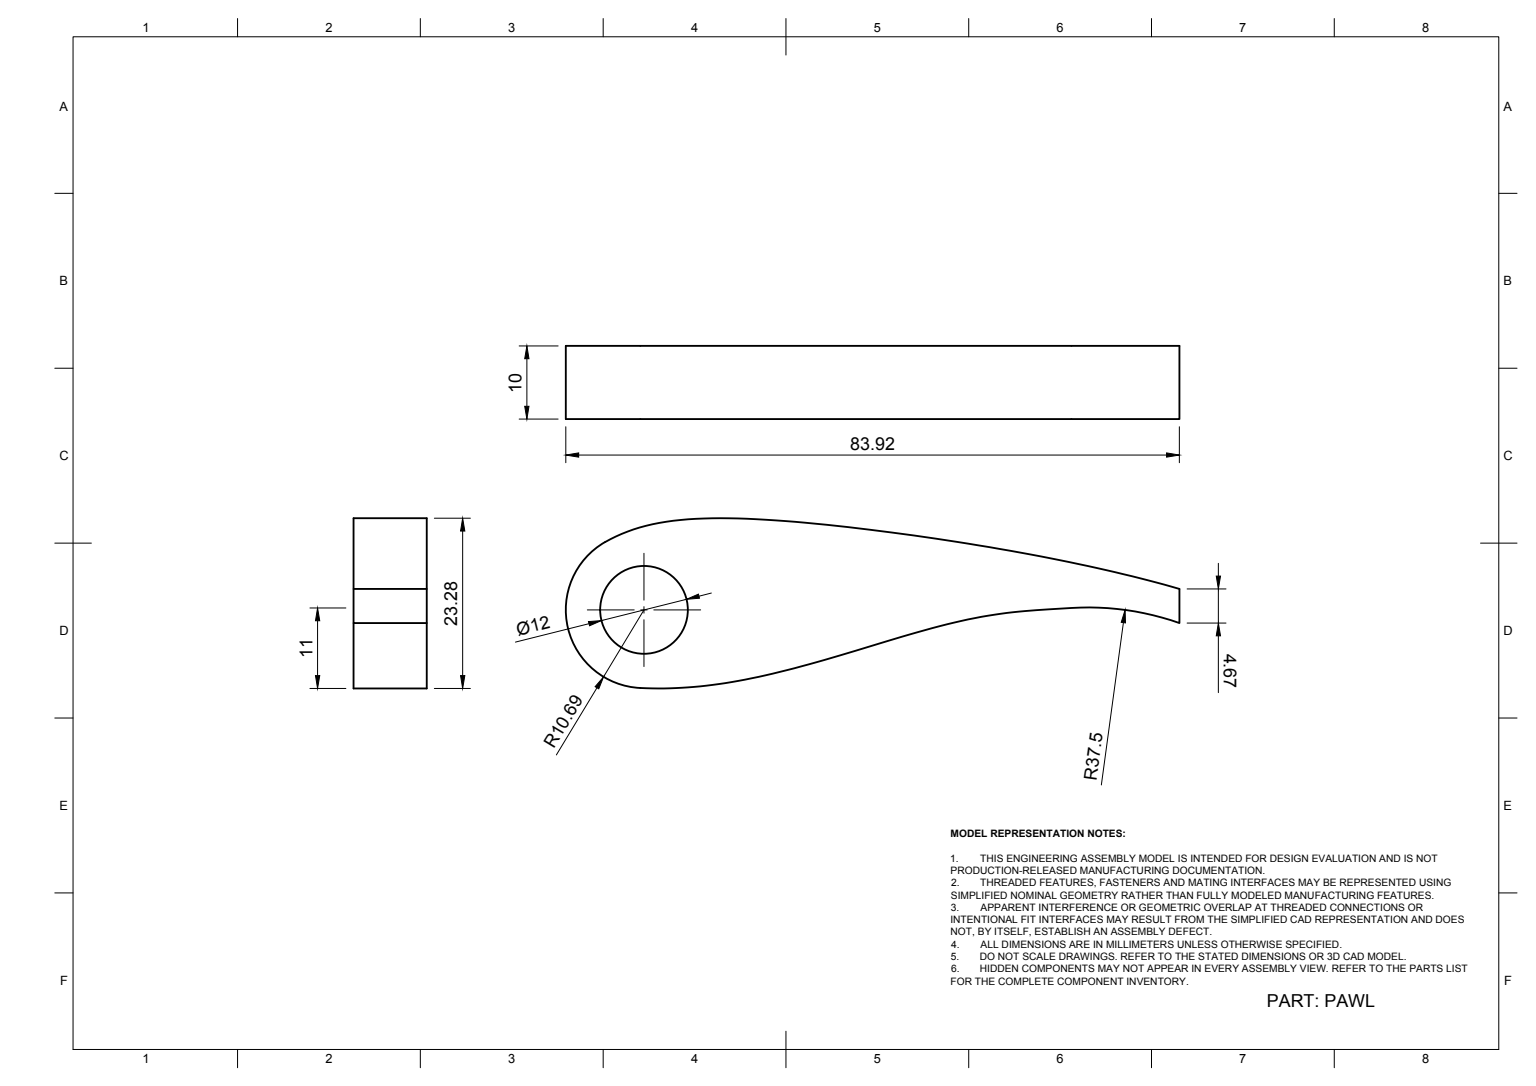
ISO-10303-21;
HEADER;
/* Generated by software containing ST-Developer
 * from STEP Tools, Inc. (www.steptools.com) 
 */

FILE_DESCRIPTION(
/* description */ (''),
/* implementation_level */ '2;1');

FILE_NAME(
/* name */ 'Pawl.step',
/* time_stamp */ '2026-09-20T22:38:01+06:00',
/* author */ (''),
/* organization */ (''),
/* preprocessor_version */ 'ST-DEVELOPER v20.2',
/* originating_system */ 'Autodesk Translation Framework v15.15.0.0',
/* authorisation */ '');

FILE_SCHEMA (('AUTOMOTIVE_DESIGN { 1 0 10303 214 3 1 1 }'));
ENDSEC;

DATA;
#10=MECHANICAL_DESIGN_GEOMETRIC_PRESENTATION_REPRESENTATION('',(#85),#4079);
#62=(
BOUNDED_CURVE()
B_SPLINE_CURVE(5,(#2402,#2403,#2404,#2405,#2406,#2407,#2408,#2409,#2410,
#2411,#2412,#2413,#2414,#2415,#2416,#2417,#2418,#2419,#2420,#2421),
 .UNSPECIFIED.,.F.,.F.)
B_SPLINE_CURVE_WITH_KNOTS((6,1,1,1,1,1,1,1,1,1,1,1,1,1,1,6),(0.,0.0666666666666667,
0.133333333333333,0.2,0.266666666666667,0.333333333333333,0.4,0.466666666666667,
0.533333333333333,0.6,0.666666666666667,0.733333333333333,0.8,0.866666666666667,
0.933333333333333,1.),.UNSPECIFIED.)
CURVE()
GEOMETRIC_REPRESENTATION_ITEM()
RATIONAL_B_SPLINE_CURVE((1.,1.,1.,1.,1.,1.,1.,1.,1.,1.,1.,1.,1.,1.,1.,1.,
1.,1.,1.,1.))
REPRESENTATION_ITEM('')
);
#63=(
BOUNDED_CURVE()
B_SPLINE_CURVE(5,(#2425,#2426,#2427,#2428,#2429,#2430,#2431,#2432,#2433,
#2434,#2435,#2436,#2437,#2438,#2439,#2440,#2441,#2442,#2443,#2444),
 .UNSPECIFIED.,.F.,.F.)
B_SPLINE_CURVE_WITH_KNOTS((6,1,1,1,1,1,1,1,1,1,1,1,1,1,1,6),(-1.,-0.933333333333333,
-0.866666666666667,-0.8,-0.733333333333333,-0.666666666666667,-0.6,-0.533333333333333,
-0.466666666666667,-0.4,-0.333333333333333,-0.266666666666667,-0.2,-0.133333333333333,
-0.0666666666666667,0.),.UNSPECIFIED.)
CURVE()
GEOMETRIC_REPRESENTATION_ITEM()
RATIONAL_B_SPLINE_CURVE((1.,1.,1.,1.,1.,1.,1.,1.,1.,1.,1.,1.,1.,1.,1.,1.,
1.,1.,1.,1.))
REPRESENTATION_ITEM('')
);
#64=(
BOUNDED_CURVE()
B_SPLINE_CURVE(5,(#2503,#2504,#2505,#2506,#2507,#2508,#2509,#2510,#2511,
#2512,#2513,#2514,#2515,#2516,#2517,#2518,#2519,#2520,#2521,#2522,#2523,
#2524,#2525,#2526,#2527),.UNSPECIFIED.,.F.,.F.)
B_SPLINE_CURVE_WITH_KNOTS((6,1,1,1,1,1,1,1,1,1,1,1,1,1,1,1,1,1,1,1,6),(0.,
0.05,0.1,0.15,0.2,0.25,0.3,0.35,0.4,0.45,0.5,0.55,0.6,0.65,0.7,0.75,0.8,
0.85,0.9,0.95,1.),.UNSPECIFIED.)
CURVE()
GEOMETRIC_REPRESENTATION_ITEM()
RATIONAL_B_SPLINE_CURVE((1.,1.,1.,1.,1.,1.,1.,1.,1.,1.,1.,1.,1.,1.,1.,1.,
1.,1.,1.,1.,1.,1.,1.,1.,1.))
REPRESENTATION_ITEM('')
);
#65=(
BOUNDED_CURVE()
B_SPLINE_CURVE(5,(#2529,#2530,#2531,#2532,#2533,#2534,#2535,#2536,#2537,
#2538,#2539,#2540,#2541,#2542,#2543,#2544,#2545,#2546,#2547,#2548,#2549,
#2550,#2551,#2552,#2553),.UNSPECIFIED.,.F.,.F.)
B_SPLINE_CURVE_WITH_KNOTS((6,1,1,1,1,1,1,1,1,1,1,1,1,1,1,1,1,1,1,1,6),(0.,
0.05,0.1,0.15,0.2,0.25,0.3,0.35,0.4,0.45,0.5,0.55,0.6,0.65,0.7,0.75,0.8,
0.85,0.9,0.95,1.),.UNSPECIFIED.)
CURVE()
GEOMETRIC_REPRESENTATION_ITEM()
RATIONAL_B_SPLINE_CURVE((1.,1.,1.,1.,1.,1.,1.,1.,1.,1.,1.,1.,1.,1.,1.,1.,
1.,1.,1.,1.,1.,1.,1.,1.,1.))
REPRESENTATION_ITEM('')
);
#66=(
BOUNDED_SURFACE()
B_SPLINE_SURFACE(5,1,((#2360,#2361),(#2362,#2363),(#2364,#2365),(#2366,
#2367),(#2368,#2369),(#2370,#2371),(#2372,#2373),(#2374,#2375),(#2376,#2377),
(#2378,#2379),(#2380,#2381),(#2382,#2383),(#2384,#2385),(#2386,#2387),(#2388,
#2389),(#2390,#2391),(#2392,#2393),(#2394,#2395),(#2396,#2397),(#2398,#2399)),
 .UNSPECIFIED.,.F.,.F.,.F.)
B_SPLINE_SURFACE_WITH_KNOTS((6,1,1,1,1,1,1,1,1,1,1,1,1,1,1,6),(2,2),(-1.,
-0.933333333333333,-0.866666666666667,-0.8,-0.733333333333333,-0.666666666666667,
-0.6,-0.533333333333333,-0.466666666666667,-0.4,-0.333333333333333,-0.266666666666667,
-0.2,-0.133333333333333,-0.0666666666666667,0.),(0.,1.),.UNSPECIFIED.)
GEOMETRIC_REPRESENTATION_ITEM()
RATIONAL_B_SPLINE_SURFACE(((1.,1.),(1.,1.),(1.,1.),(1.,1.),(1.,1.),(1.,
1.),(1.,1.),(1.,1.),(1.,1.),(1.,1.),(1.,1.),(1.,1.),(1.,1.),(1.,1.),(1.,
1.),(1.,1.),(1.,1.),(1.,1.),(1.,1.),(1.,1.)))
REPRESENTATION_ITEM('')
SURFACE()
);
#67=(
BOUNDED_SURFACE()
B_SPLINE_SURFACE(5,1,((#2452,#2453),(#2454,#2455),(#2456,#2457),(#2458,
#2459),(#2460,#2461),(#2462,#2463),(#2464,#2465),(#2466,#2467),(#2468,#2469),
(#2470,#2471),(#2472,#2473),(#2474,#2475),(#2476,#2477),(#2478,#2479),(#2480,
#2481),(#2482,#2483),(#2484,#2485),(#2486,#2487),(#2488,#2489),(#2490,#2491),
(#2492,#2493),(#2494,#2495),(#2496,#2497),(#2498,#2499),(#2500,#2501)),
 .UNSPECIFIED.,.F.,.F.,.F.)
B_SPLINE_SURFACE_WITH_KNOTS((6,1,1,1,1,1,1,1,1,1,1,1,1,1,1,1,1,1,1,1,6),
(2,2),(0.,0.05,0.1,0.15,0.2,0.25,0.3,0.35,0.4,0.45,0.5,0.55,0.6,0.65,0.7,
0.75,0.8,0.85,0.9,0.95,1.),(0.,1.),.UNSPECIFIED.)
GEOMETRIC_REPRESENTATION_ITEM()
RATIONAL_B_SPLINE_SURFACE(((1.,1.),(1.,1.),(1.,1.),(1.,1.),(1.,1.),(1.,
1.),(1.,1.),(1.,1.),(1.,1.),(1.,1.),(1.,1.),(1.,1.),(1.,1.),(1.,1.),(1.,
1.),(1.,1.),(1.,1.),(1.,1.),(1.,1.),(1.,1.),(1.,1.),(1.,1.),(1.,1.),(1.,
1.),(1.,1.)))
REPRESENTATION_ITEM('')
SURFACE()
);
#69=SHAPE_REPRESENTATION_RELATIONSHIP('SRR','None',#4112,#77);
#77=ADVANCED_BREP_SHAPE_REPRESENTATION('',(#93),#4072);
#85=STYLED_ITEM('',(#4161),#93);
#93=MANIFOLD_SOLID_BREP('Pawl',#1444);
#102=FACE_BOUND('',#329,.T.);
#103=FACE_BOUND('',#331,.T.);
#144=CIRCLE('',#1621,6.);
#145=CIRCLE('',#1622,6.);
#146=CIRCLE('',#1624,10.6886401797172);
#147=CIRCLE('',#1625,10.6886401797172);
#148=CIRCLE('',#1627,37.4987147312738);
#149=CIRCLE('',#1628,37.4987147312738);
#188=CYLINDRICAL_SURFACE('',#1620,6.);
#189=CYLINDRICAL_SURFACE('',#1623,10.6886401797172);
#190=CYLINDRICAL_SURFACE('',#1626,37.4987147312738);
#236=FACE_OUTER_BOUND('',#322,.T.);
#237=FACE_OUTER_BOUND('',#323,.T.);
#238=FACE_OUTER_BOUND('',#324,.T.);
#239=FACE_OUTER_BOUND('',#325,.T.);
#240=FACE_OUTER_BOUND('',#326,.T.);
#241=FACE_OUTER_BOUND('',#327,.T.);
#242=FACE_OUTER_BOUND('',#328,.T.);
#243=FACE_OUTER_BOUND('',#330,.T.);
#322=EDGE_LOOP('',(#1141,#1142,#1143,#1144));
#323=EDGE_LOOP('',(#1145,#1146,#1147,#1148));
#324=EDGE_LOOP('',(#1149,#1150,#1151,#1152));
#325=EDGE_LOOP('',(#1153,#1154,#1155,#1156));
#326=EDGE_LOOP('',(#1157,#1158,#1159,#1160));
#327=EDGE_LOOP('',(#1161,#1162,#1163,#1164));
#328=EDGE_LOOP('',(#1165,#1166,#1167,#1168,#1169));
#329=EDGE_LOOP('',(#1170));
#330=EDGE_LOOP('',(#1171,#1172,#1173,#1174,#1175));
#331=EDGE_LOOP('',(#1176));
#444=LINE('',#2358,#557);
#445=LINE('',#2423,#558);
#446=LINE('',#2445,#559);
#447=LINE('',#2451,#560);
#448=LINE('',#2554,#561);
#449=LINE('',#2560,#562);
#450=LINE('',#2562,#563);
#451=LINE('',#2563,#564);
#557=VECTOR('',#1935,6.);
#558=VECTOR('',#1938,10.);
#559=VECTOR('',#1939,10.);
#560=VECTOR('',#1946,10.);
#561=VECTOR('',#1947,10.);
#562=VECTOR('',#1954,10.);
#563=VECTOR('',#1957,10.);
#564=VECTOR('',#1958,10.);
#671=VERTEX_POINT('',#2355);
#672=VERTEX_POINT('',#2357);
#673=VERTEX_POINT('',#2400);
#674=VERTEX_POINT('',#2401);
#675=VERTEX_POINT('',#2422);
#676=VERTEX_POINT('',#2424);
#677=VERTEX_POINT('',#2447);
#678=VERTEX_POINT('',#2449);
#679=VERTEX_POINT('',#2502);
#680=VERTEX_POINT('',#2528);
#681=VERTEX_POINT('',#2556);
#682=VERTEX_POINT('',#2558);
#835=EDGE_CURVE('',#671,#671,#144,.T.);
#836=EDGE_CURVE('',#671,#672,#444,.T.);
#837=EDGE_CURVE('',#672,#672,#145,.T.);
#838=EDGE_CURVE('',#673,#674,#62,.T.);
#839=EDGE_CURVE('',#673,#675,#445,.T.);
#840=EDGE_CURVE('',#676,#675,#63,.T.);
#841=EDGE_CURVE('',#674,#676,#446,.T.);
#842=EDGE_CURVE('',#674,#677,#146,.T.);
#843=EDGE_CURVE('',#678,#676,#147,.T.);
#844=EDGE_CURVE('',#677,#678,#447,.T.);
#845=EDGE_CURVE('',#679,#677,#64,.T.);
#846=EDGE_CURVE('',#680,#678,#65,.T.);
#847=EDGE_CURVE('',#679,#680,#448,.T.);
#848=EDGE_CURVE('',#681,#679,#148,.T.);
#849=EDGE_CURVE('',#682,#680,#149,.T.);
#850=EDGE_CURVE('',#681,#682,#449,.T.);
#851=EDGE_CURVE('',#681,#673,#450,.T.);
#852=EDGE_CURVE('',#675,#682,#451,.T.);
#1141=ORIENTED_EDGE('',*,*,#835,.F.);
#1142=ORIENTED_EDGE('',*,*,#836,.T.);
#1143=ORIENTED_EDGE('',*,*,#837,.F.);
#1144=ORIENTED_EDGE('',*,*,#836,.F.);
#1145=ORIENTED_EDGE('',*,*,#838,.F.);
#1146=ORIENTED_EDGE('',*,*,#839,.T.);
#1147=ORIENTED_EDGE('',*,*,#840,.F.);
#1148=ORIENTED_EDGE('',*,*,#841,.F.);
#1149=ORIENTED_EDGE('',*,*,#842,.F.);
#1150=ORIENTED_EDGE('',*,*,#841,.T.);
#1151=ORIENTED_EDGE('',*,*,#843,.F.);
#1152=ORIENTED_EDGE('',*,*,#844,.F.);
#1153=ORIENTED_EDGE('',*,*,#845,.T.);
#1154=ORIENTED_EDGE('',*,*,#844,.T.);
#1155=ORIENTED_EDGE('',*,*,#846,.F.);
#1156=ORIENTED_EDGE('',*,*,#847,.F.);
#1157=ORIENTED_EDGE('',*,*,#848,.T.);
#1158=ORIENTED_EDGE('',*,*,#847,.T.);
#1159=ORIENTED_EDGE('',*,*,#849,.F.);
#1160=ORIENTED_EDGE('',*,*,#850,.F.);
#1161=ORIENTED_EDGE('',*,*,#851,.F.);
#1162=ORIENTED_EDGE('',*,*,#850,.T.);
#1163=ORIENTED_EDGE('',*,*,#852,.F.);
#1164=ORIENTED_EDGE('',*,*,#839,.F.);
#1165=ORIENTED_EDGE('',*,*,#851,.T.);
#1166=ORIENTED_EDGE('',*,*,#838,.T.);
#1167=ORIENTED_EDGE('',*,*,#842,.T.);
#1168=ORIENTED_EDGE('',*,*,#845,.F.);
#1169=ORIENTED_EDGE('',*,*,#848,.F.);
#1170=ORIENTED_EDGE('',*,*,#835,.T.);
#1171=ORIENTED_EDGE('',*,*,#852,.T.);
#1172=ORIENTED_EDGE('',*,*,#849,.T.);
#1173=ORIENTED_EDGE('',*,*,#846,.T.);
#1174=ORIENTED_EDGE('',*,*,#843,.T.);
#1175=ORIENTED_EDGE('',*,*,#840,.T.);
#1176=ORIENTED_EDGE('',*,*,#837,.T.);
#1329=PLANE('',#1629);
#1330=PLANE('',#1630);
#1331=PLANE('',#1631);
#1398=ADVANCED_FACE('',(#236),#188,.F.);
#1399=ADVANCED_FACE('',(#237),#66,.T.);
#1400=ADVANCED_FACE('',(#238),#189,.T.);
#1401=ADVANCED_FACE('',(#239),#67,.T.);
#1402=ADVANCED_FACE('',(#240),#190,.F.);
#1403=ADVANCED_FACE('',(#241),#1329,.T.);
#1404=ADVANCED_FACE('',(#242,#102),#1330,.T.);
#1405=ADVANCED_FACE('',(#243,#103),#1331,.F.);
#1444=CLOSED_SHELL('',(#1398,#1399,#1400,#1401,#1402,#1403,#1404,#1405));
#1619=AXIS2_PLACEMENT_3D('',#2353,#1929,#1930);
#1620=AXIS2_PLACEMENT_3D('',#2354,#1931,#1932);
#1621=AXIS2_PLACEMENT_3D('',#2356,#1933,#1934);
#1622=AXIS2_PLACEMENT_3D('',#2359,#1936,#1937);
#1623=AXIS2_PLACEMENT_3D('',#2446,#1940,#1941);
#1624=AXIS2_PLACEMENT_3D('',#2448,#1942,#1943);
#1625=AXIS2_PLACEMENT_3D('',#2450,#1944,#1945);
#1626=AXIS2_PLACEMENT_3D('',#2555,#1948,#1949);
#1627=AXIS2_PLACEMENT_3D('',#2557,#1950,#1951);
#1628=AXIS2_PLACEMENT_3D('',#2559,#1952,#1953);
#1629=AXIS2_PLACEMENT_3D('',#2561,#1955,#1956);
#1630=AXIS2_PLACEMENT_3D('',#2564,#1959,#1960);
#1631=AXIS2_PLACEMENT_3D('',#2565,#1961,#1962);
#1929=DIRECTION('axis',(0.,0.,1.));
#1930=DIRECTION('refdir',(1.,0.,0.));
#1931=DIRECTION('center_axis',(0.,-1.,0.));
#1932=DIRECTION('ref_axis',(1.,0.,0.));
#1933=DIRECTION('center_axis',(0.,-1.,0.));
#1934=DIRECTION('ref_axis',(1.,0.,0.));
#1935=DIRECTION('',(0.,-1.,0.));
#1936=DIRECTION('center_axis',(0.,1.,0.));
#1937=DIRECTION('ref_axis',(1.,0.,0.));
#1938=DIRECTION('',(0.,-1.,0.));
#1939=DIRECTION('',(0.,-1.,0.));
#1940=DIRECTION('center_axis',(0.,-1.,0.));
#1941=DIRECTION('ref_axis',(1.,0.,0.));
#1942=DIRECTION('center_axis',(0.,1.,0.));
#1943=DIRECTION('ref_axis',(1.,0.,0.));
#1944=DIRECTION('center_axis',(0.,-1.,0.));
#1945=DIRECTION('ref_axis',(1.,0.,0.));
#1946=DIRECTION('',(0.,-1.,0.));
#1947=DIRECTION('',(0.,-1.,0.));
#1948=DIRECTION('center_axis',(0.,-1.,0.));
#1949=DIRECTION('ref_axis',(-0.332459503726204,0.,0.943117531584546));
#1950=DIRECTION('center_axis',(0.,1.,0.));
#1951=DIRECTION('ref_axis',(-0.332459503726204,0.,0.943117531584546));
#1952=DIRECTION('center_axis',(0.,1.,0.));
#1953=DIRECTION('ref_axis',(-0.332459503726204,0.,0.943117531584546));
#1954=DIRECTION('',(0.,-1.,0.));
#1955=DIRECTION('center_axis',(-0.999999995604207,0.,9.37634563086646E-5));
#1956=DIRECTION('ref_axis',(-9.37634563086646E-5,0.,-0.999999995604207));
#1957=DIRECTION('',(9.37634563086646E-5,0.,0.999999995604207));
#1958=DIRECTION('',(-9.37634563086646E-5,0.,-0.999999995604207));
#1959=DIRECTION('center_axis',(0.,1.,0.));
#1960=DIRECTION('ref_axis',(1.,0.,0.));
#1961=DIRECTION('center_axis',(0.,1.,0.));
#1962=DIRECTION('ref_axis',(1.,0.,0.));
#2353=CARTESIAN_POINT('',(0.,0.,0.));
#2354=CARTESIAN_POINT('Origin',(73.2288574389116,0.,87.4952777324745));
#2355=CARTESIAN_POINT('',(67.2288574389116,0.,87.4952777324745));
#2356=CARTESIAN_POINT('Origin',(73.2288574389116,0.,87.4952777324745));
#2357=CARTESIAN_POINT('',(67.2288574389116,-10.,87.4952777324745));
#2358=CARTESIAN_POINT('',(67.2288574389116,0.,87.4952777324745));
#2359=CARTESIAN_POINT('Origin',(73.2288574389116,-10.,87.4952777324745));
#2360=CARTESIAN_POINT('Ctrl Pts',(78.5565765069325,0.,96.7614764365663));
#2361=CARTESIAN_POINT('Ctrl Pts',(78.5565765069325,-10.,96.7614764365663));
#2362=CARTESIAN_POINT('Ctrl Pts',(77.933781500681,0.,97.1195603646402));
#2363=CARTESIAN_POINT('Ctrl Pts',(77.933781500681,-10.,97.1195603646402));
#2364=CARTESIAN_POINT('Ctrl Pts',(76.6526666483233,0.,97.7826386838039));
#2365=CARTESIAN_POINT('Ctrl Pts',(76.6526666483233,-10.,97.7826386838039));
#2366=CARTESIAN_POINT('Ctrl Pts',(74.6244214366979,0.,98.6179893838346));
#2367=CARTESIAN_POINT('Ctrl Pts',(74.6244214366979,-10.,98.6179893838346));
#2368=CARTESIAN_POINT('Ctrl Pts',(71.6890880153669,0.,99.4224704752722));
#2369=CARTESIAN_POINT('Ctrl Pts',(71.6890880153669,-10.,99.4224704752722));
#2370=CARTESIAN_POINT('Ctrl Pts',(67.5475314586935,0.,99.9655376285179));
#2371=CARTESIAN_POINT('Ctrl Pts',(67.5475314586935,-10.,99.9655376285179));
#2372=CARTESIAN_POINT('Ctrl Pts',(62.8494346176935,0.,100.11488638886));
#2373=CARTESIAN_POINT('Ctrl Pts',(62.8494346176935,-10.,100.11488638886));
#2374=CARTESIAN_POINT('Ctrl Pts',(57.5623233061826,0.,99.9423456500588));
#2375=CARTESIAN_POINT('Ctrl Pts',(57.5623233061826,-10.,99.9423456500588));
#2376=CARTESIAN_POINT('Ctrl Pts',(51.7530480696311,0.,99.5113992758897));
#2377=CARTESIAN_POINT('Ctrl Pts',(51.7530480696311,-10.,99.5113992758897));
#2378=CARTESIAN_POINT('Ctrl Pts',(45.5547012575949,0.,98.8769393338912));
#2379=CARTESIAN_POINT('Ctrl Pts',(45.5547012575949,-10.,98.8769393338912));
#2380=CARTESIAN_POINT('Ctrl Pts',(39.1395829757266,0.,98.0850994498989));
#2381=CARTESIAN_POINT('Ctrl Pts',(39.1395829757266,-10.,98.0850994498989));
#2382=CARTESIAN_POINT('Ctrl Pts',(32.6920975126609,0.,97.1735392968004));
#2383=CARTESIAN_POINT('Ctrl Pts',(32.6920975126609,-10.,97.1735392968004));
#2384=CARTESIAN_POINT('Ctrl Pts',(26.384627993242,0.,96.1718956743097));
#2385=CARTESIAN_POINT('Ctrl Pts',(26.384627993242,-10.,96.1718956743097));
#2386=CARTESIAN_POINT('Ctrl Pts',(20.3489626390195,0.,95.1023403943181));
#2387=CARTESIAN_POINT('Ctrl Pts',(20.3489626390195,-10.,95.1023403943181));
#2388=CARTESIAN_POINT('Ctrl Pts',(14.6587606984742,0.,93.9803229433208));
#2389=CARTESIAN_POINT('Ctrl Pts',(14.6587606984742,-10.,93.9803229433208));
#2390=CARTESIAN_POINT('Ctrl Pts',(9.3499076568271,0.,92.8157760857789));
#2391=CARTESIAN_POINT('Ctrl Pts',(9.3499076568271,-10.,92.8157760857789));
#2392=CARTESIAN_POINT('Ctrl Pts',(5.41600698566024,0.,91.854562206062));
#2393=CARTESIAN_POINT('Ctrl Pts',(5.41600698566024,-10.,91.854562206062));
#2394=CARTESIAN_POINT('Ctrl Pts',(2.64064416187385,0.,91.1180813473512));
#2395=CARTESIAN_POINT('Ctrl Pts',(2.64064416187385,-10.,91.1180813473512));
#2396=CARTESIAN_POINT('Ctrl Pts',(0.867636945837178,0.,90.6202239141436));
#2397=CARTESIAN_POINT('Ctrl Pts',(0.867636945837178,-10.,90.6202239141436));
#2398=CARTESIAN_POINT('Ctrl Pts',(0.000442544535028507,0.,90.3695776431675));
#2399=CARTESIAN_POINT('Ctrl Pts',(0.000442544535028507,-10.,90.3695776431675));
#2400=CARTESIAN_POINT('',(0.000442544535028507,0.,90.3695776431675));
#2401=CARTESIAN_POINT('',(78.5565765069325,0.,96.7614764365663));
#2402=CARTESIAN_POINT('Ctrl Pts',(0.000442544535028507,0.,90.3695776431675));
#2403=CARTESIAN_POINT('Ctrl Pts',(0.867636945837178,0.,90.6202239141436));
#2404=CARTESIAN_POINT('Ctrl Pts',(2.64064416187385,0.,91.1180813473512));
#2405=CARTESIAN_POINT('Ctrl Pts',(5.41600698566024,0.,91.854562206062));
#2406=CARTESIAN_POINT('Ctrl Pts',(9.3499076568271,0.,92.8157760857789));
#2407=CARTESIAN_POINT('Ctrl Pts',(14.6587606984742,0.,93.9803229433208));
#2408=CARTESIAN_POINT('Ctrl Pts',(20.3489626390195,0.,95.1023403943181));
#2409=CARTESIAN_POINT('Ctrl Pts',(26.384627993242,0.,96.1718956743097));
#2410=CARTESIAN_POINT('Ctrl Pts',(32.6920975126609,0.,97.1735392968004));
#2411=CARTESIAN_POINT('Ctrl Pts',(39.1395829757266,0.,98.0850994498989));
#2412=CARTESIAN_POINT('Ctrl Pts',(45.5547012575949,0.,98.8769393338912));
#2413=CARTESIAN_POINT('Ctrl Pts',(51.7530480696311,0.,99.5113992758897));
#2414=CARTESIAN_POINT('Ctrl Pts',(57.5623233061826,0.,99.9423456500588));
#2415=CARTESIAN_POINT('Ctrl Pts',(62.8494346176935,0.,100.11488638886));
#2416=CARTESIAN_POINT('Ctrl Pts',(67.5475314586935,0.,99.9655376285179));
#2417=CARTESIAN_POINT('Ctrl Pts',(71.6890880153669,0.,99.4224704752722));
#2418=CARTESIAN_POINT('Ctrl Pts',(74.6244214366979,0.,98.6179893838346));
#2419=CARTESIAN_POINT('Ctrl Pts',(76.6526666483233,0.,97.7826386838039));
#2420=CARTESIAN_POINT('Ctrl Pts',(77.933781500681,0.,97.1195603646402));
#2421=CARTESIAN_POINT('Ctrl Pts',(78.5565765069325,0.,96.7614764365663));
#2422=CARTESIAN_POINT('',(0.000442544535028507,-10.,90.3695776431675));
#2423=CARTESIAN_POINT('',(0.000442544535028507,0.,90.3695776431675));
#2424=CARTESIAN_POINT('',(78.5565765069325,-10.,96.7614764365663));
#2425=CARTESIAN_POINT('Ctrl Pts',(78.5565765069325,-10.,96.7614764365663));
#2426=CARTESIAN_POINT('Ctrl Pts',(77.933781500681,-10.,97.1195603646402));
#2427=CARTESIAN_POINT('Ctrl Pts',(76.6526666483233,-10.,97.7826386838039));
#2428=CARTESIAN_POINT('Ctrl Pts',(74.6244214366979,-10.,98.6179893838346));
#2429=CARTESIAN_POINT('Ctrl Pts',(71.6890880153669,-10.,99.4224704752722));
#2430=CARTESIAN_POINT('Ctrl Pts',(67.5475314586935,-10.,99.9655376285179));
#2431=CARTESIAN_POINT('Ctrl Pts',(62.8494346176935,-10.,100.11488638886));
#2432=CARTESIAN_POINT('Ctrl Pts',(57.5623233061826,-10.,99.9423456500588));
#2433=CARTESIAN_POINT('Ctrl Pts',(51.7530480696311,-10.,99.5113992758897));
#2434=CARTESIAN_POINT('Ctrl Pts',(45.5547012575949,-10.,98.8769393338912));
#2435=CARTESIAN_POINT('Ctrl Pts',(39.1395829757266,-10.,98.0850994498989));
#2436=CARTESIAN_POINT('Ctrl Pts',(32.6920975126609,-10.,97.1735392968004));
#2437=CARTESIAN_POINT('Ctrl Pts',(26.384627993242,-10.,96.1718956743097));
#2438=CARTESIAN_POINT('Ctrl Pts',(20.3489626390195,-10.,95.1023403943181));
#2439=CARTESIAN_POINT('Ctrl Pts',(14.6587606984742,-10.,93.9803229433208));
#2440=CARTESIAN_POINT('Ctrl Pts',(9.3499076568271,-10.,92.8157760857789));
#2441=CARTESIAN_POINT('Ctrl Pts',(5.41600698566024,-10.,91.854562206062));
#2442=CARTESIAN_POINT('Ctrl Pts',(2.64064416187385,-10.,91.1180813473512));
#2443=CARTESIAN_POINT('Ctrl Pts',(0.867636945837178,-10.,90.6202239141436));
#2444=CARTESIAN_POINT('Ctrl Pts',(0.000442544535028507,-10.,90.3695776431675));
#2445=CARTESIAN_POINT('',(78.5565765069325,0.,96.7614764365663));
#2446=CARTESIAN_POINT('Origin',(73.2288574389116,0.,87.4952777324745));
#2447=CARTESIAN_POINT('',(73.7249441578369,0.,76.8181560763928));
#2448=CARTESIAN_POINT('Origin',(73.2288574389116,0.,87.4952777324745));
#2449=CARTESIAN_POINT('',(73.7249441578369,-10.,76.8181560763928));
#2450=CARTESIAN_POINT('Origin',(73.2288574389116,-10.,87.4952777324745));
#2451=CARTESIAN_POINT('',(73.7249441578369,0.,76.8181560763928));
#2452=CARTESIAN_POINT('Ctrl Pts',(14.7760680196183,0.,87.7628077035488));
#2453=CARTESIAN_POINT('Ctrl Pts',(14.7760680196183,-10.,87.7628077035488));
#2454=CARTESIAN_POINT('Ctrl Pts',(15.2822994559612,0.,87.7315734976063));
#2455=CARTESIAN_POINT('Ctrl Pts',(15.2822994559612,-10.,87.7315734976063));
#2456=CARTESIAN_POINT('Ctrl Pts',(16.2934759211885,0.,87.669785304704));
#2457=CARTESIAN_POINT('Ctrl Pts',(16.2934759211885,-10.,87.669785304704));
#2458=CARTESIAN_POINT('Ctrl Pts',(17.8063864959714,0.,87.5791386198598));
#2459=CARTESIAN_POINT('Ctrl Pts',(17.8063864959714,-10.,87.5791386198598));
#2460=CARTESIAN_POINT('Ctrl Pts',(19.8250496559672,0.,87.4534593828614));
#2461=CARTESIAN_POINT('Ctrl Pts',(19.8250496559672,-10.,87.4534593828614));
#2462=CARTESIAN_POINT('Ctrl Pts',(22.4011592565578,0.,87.2395858399089));
#2463=CARTESIAN_POINT('Ctrl Pts',(22.4011592565578,-10.,87.2395858399089));
#2464=CARTESIAN_POINT('Ctrl Pts',(25.0887629856102,0.,86.9124001611246));
#2465=CARTESIAN_POINT('Ctrl Pts',(25.0887629856102,-10.,86.9124001611246));
#2466=CARTESIAN_POINT('Ctrl Pts',(27.9380040884934,0.,86.4241239702294));
#2467=CARTESIAN_POINT('Ctrl Pts',(27.9380040884934,-10.,86.4241239702294));
#2468=CARTESIAN_POINT('Ctrl Pts',(30.9683248537247,0.,85.75747543975));
#2469=CARTESIAN_POINT('Ctrl Pts',(30.9683248537247,-10.,85.75747543975));
#2470=CARTESIAN_POINT('Ctrl Pts',(34.165400944085,0.,84.928453366817));
#2471=CARTESIAN_POINT('Ctrl Pts',(34.165400944085,-10.,84.928453366817));
#2472=CARTESIAN_POINT('Ctrl Pts',(37.4932382987616,0.,83.9740394198894));
#2473=CARTESIAN_POINT('Ctrl Pts',(37.4932382987616,-10.,83.9740394198894));
#2474=CARTESIAN_POINT('Ctrl Pts',(40.9013700189392,0.,82.9447683400012));
#2475=CARTESIAN_POINT('Ctrl Pts',(40.9013700189392,-10.,82.9447683400012));
#2476=CARTESIAN_POINT('Ctrl Pts',(44.3336493923615,0.,81.8956839784984));
#2477=CARTESIAN_POINT('Ctrl Pts',(44.3336493923615,-10.,81.8956839784984));
#2478=CARTESIAN_POINT('Ctrl Pts',(47.7360606768338,0.,80.8782861138939));
#2479=CARTESIAN_POINT('Ctrl Pts',(47.7360606768338,-10.,80.8782861138939));
#2480=CARTESIAN_POINT('Ctrl Pts',(51.0650378422273,0.,79.9318697713207));
#2481=CARTESIAN_POINT('Ctrl Pts',(51.0650378422273,-10.,79.9318697713207));
#2482=CARTESIAN_POINT('Ctrl Pts',(54.288048859871,0.,79.085110401947));
#2483=CARTESIAN_POINT('Ctrl Pts',(54.288048859871,-10.,79.085110401947));
#2484=CARTESIAN_POINT('Ctrl Pts',(57.3840999328369,0.,78.357680633469));
#2485=CARTESIAN_POINT('Ctrl Pts',(57.3840999328369,-10.,78.357680633469));
#2486=CARTESIAN_POINT('Ctrl Pts',(60.3448286085174,0.,77.7615650133373));
#2487=CARTESIAN_POINT('Ctrl Pts',(60.3448286085174,-10.,77.7615650133373));
#2488=CARTESIAN_POINT('Ctrl Pts',(63.175078635463,0.,77.3023279219762));
#2489=CARTESIAN_POINT('Ctrl Pts',(63.175078635463,-10.,77.3023279219762));
#2490=CARTESIAN_POINT('Ctrl Pts',(65.8955912826513,0.,76.9799168209156));
#2491=CARTESIAN_POINT('Ctrl Pts',(65.8955912826513,-10.,76.9799168209156));
#2492=CARTESIAN_POINT('Ctrl Pts',(68.5390245353947,0.,76.7903239063253));
#2493=CARTESIAN_POINT('Ctrl Pts',(68.5390245353947,-10.,76.7903239063253));
#2494=CARTESIAN_POINT('Ctrl Pts',(70.619638872722,0.,76.7404944287697));
#2495=CARTESIAN_POINT('Ctrl Pts',(70.619638872722,-10.,76.7404944287697));
#2496=CARTESIAN_POINT('Ctrl Pts',(72.1734485372099,0.,76.7581820414634));
#2497=CARTESIAN_POINT('Ctrl Pts',(72.1734485372099,-10.,76.7581820414634));
#2498=CARTESIAN_POINT('Ctrl Pts',(73.2079991529442,0.,76.7941374729149));
#2499=CARTESIAN_POINT('Ctrl Pts',(73.2079991529442,-10.,76.7941374729149));
#2500=CARTESIAN_POINT('Ctrl Pts',(73.7249441578369,0.,76.8181560763928));
#2501=CARTESIAN_POINT('Ctrl Pts',(73.7249441578369,-10.,76.8181560763928));
#2502=CARTESIAN_POINT('',(14.7760680196183,0.,87.7628077035488));
#2503=CARTESIAN_POINT('Ctrl Pts',(14.7760680196183,0.,87.7628077035488));
#2504=CARTESIAN_POINT('Ctrl Pts',(15.2822994559612,0.,87.7315734976063));
#2505=CARTESIAN_POINT('Ctrl Pts',(16.2934759211885,0.,87.669785304704));
#2506=CARTESIAN_POINT('Ctrl Pts',(17.8063864959714,0.,87.5791386198598));
#2507=CARTESIAN_POINT('Ctrl Pts',(19.8250496559672,0.,87.4534593828614));
#2508=CARTESIAN_POINT('Ctrl Pts',(22.4011592565578,0.,87.2395858399089));
#2509=CARTESIAN_POINT('Ctrl Pts',(25.0887629856102,0.,86.9124001611246));
#2510=CARTESIAN_POINT('Ctrl Pts',(27.9380040884934,0.,86.4241239702294));
#2511=CARTESIAN_POINT('Ctrl Pts',(30.9683248537247,0.,85.75747543975));
#2512=CARTESIAN_POINT('Ctrl Pts',(34.165400944085,0.,84.928453366817));
#2513=CARTESIAN_POINT('Ctrl Pts',(37.4932382987616,0.,83.9740394198894));
#2514=CARTESIAN_POINT('Ctrl Pts',(40.9013700189392,0.,82.9447683400012));
#2515=CARTESIAN_POINT('Ctrl Pts',(44.3336493923615,0.,81.8956839784984));
#2516=CARTESIAN_POINT('Ctrl Pts',(47.7360606768338,0.,80.8782861138939));
#2517=CARTESIAN_POINT('Ctrl Pts',(51.0650378422273,0.,79.9318697713207));
#2518=CARTESIAN_POINT('Ctrl Pts',(54.288048859871,0.,79.085110401947));
#2519=CARTESIAN_POINT('Ctrl Pts',(57.3840999328369,0.,78.357680633469));
#2520=CARTESIAN_POINT('Ctrl Pts',(60.3448286085174,0.,77.7615650133373));
#2521=CARTESIAN_POINT('Ctrl Pts',(63.175078635463,0.,77.3023279219762));
#2522=CARTESIAN_POINT('Ctrl Pts',(65.8955912826513,0.,76.9799168209156));
#2523=CARTESIAN_POINT('Ctrl Pts',(68.5390245353947,0.,76.7903239063253));
#2524=CARTESIAN_POINT('Ctrl Pts',(70.619638872722,0.,76.7404944287697));
#2525=CARTESIAN_POINT('Ctrl Pts',(72.1734485372099,0.,76.7581820414634));
#2526=CARTESIAN_POINT('Ctrl Pts',(73.2079991529442,0.,76.7941374729149));
#2527=CARTESIAN_POINT('Ctrl Pts',(73.7249441578369,0.,76.8181560763928));
#2528=CARTESIAN_POINT('',(14.7760680196183,-10.,87.7628077035488));
#2529=CARTESIAN_POINT('Ctrl Pts',(14.7760680196183,-10.,87.7628077035488));
#2530=CARTESIAN_POINT('Ctrl Pts',(15.2822994559612,-10.,87.7315734976063));
#2531=CARTESIAN_POINT('Ctrl Pts',(16.2934759211885,-10.,87.669785304704));
#2532=CARTESIAN_POINT('Ctrl Pts',(17.8063864959714,-10.,87.5791386198598));
#2533=CARTESIAN_POINT('Ctrl Pts',(19.8250496559672,-10.,87.4534593828614));
#2534=CARTESIAN_POINT('Ctrl Pts',(22.4011592565578,-10.,87.2395858399089));
#2535=CARTESIAN_POINT('Ctrl Pts',(25.0887629856102,-10.,86.9124001611246));
#2536=CARTESIAN_POINT('Ctrl Pts',(27.9380040884934,-10.,86.4241239702294));
#2537=CARTESIAN_POINT('Ctrl Pts',(30.9683248537247,-10.,85.75747543975));
#2538=CARTESIAN_POINT('Ctrl Pts',(34.165400944085,-10.,84.928453366817));
#2539=CARTESIAN_POINT('Ctrl Pts',(37.4932382987616,-10.,83.9740394198894));
#2540=CARTESIAN_POINT('Ctrl Pts',(40.9013700189392,-10.,82.9447683400012));
#2541=CARTESIAN_POINT('Ctrl Pts',(44.3336493923615,-10.,81.8956839784984));
#2542=CARTESIAN_POINT('Ctrl Pts',(47.7360606768338,-10.,80.8782861138939));
#2543=CARTESIAN_POINT('Ctrl Pts',(51.0650378422273,-10.,79.9318697713207));
#2544=CARTESIAN_POINT('Ctrl Pts',(54.288048859871,-10.,79.085110401947));
#2545=CARTESIAN_POINT('Ctrl Pts',(57.3840999328369,-10.,78.357680633469));
#2546=CARTESIAN_POINT('Ctrl Pts',(60.3448286085174,-10.,77.7615650133373));
#2547=CARTESIAN_POINT('Ctrl Pts',(63.175078635463,-10.,77.3023279219762));
#2548=CARTESIAN_POINT('Ctrl Pts',(65.8955912826513,-10.,76.9799168209156));
#2549=CARTESIAN_POINT('Ctrl Pts',(68.5390245353947,-10.,76.7903239063253));
#2550=CARTESIAN_POINT('Ctrl Pts',(70.619638872722,-10.,76.7404944287697));
#2551=CARTESIAN_POINT('Ctrl Pts',(72.1734485372099,-10.,76.7581820414634));
#2552=CARTESIAN_POINT('Ctrl Pts',(73.2079991529442,-10.,76.7941374729149));
#2553=CARTESIAN_POINT('Ctrl Pts',(73.7249441578369,-10.,76.8181560763928));
#2554=CARTESIAN_POINT('',(14.7760680196183,0.,87.7628077035488));
#2555=CARTESIAN_POINT('Origin',(12.4668088887924,0.,50.3352653214454));
#2556=CARTESIAN_POINT('',(4.79886262727547E-6,0.,85.7009605963974));
#2557=CARTESIAN_POINT('Origin',(12.4668088887924,0.,50.3352653214454));
#2558=CARTESIAN_POINT('',(4.79886262727547E-6,-10.,85.7009605963974));
#2559=CARTESIAN_POINT('Origin',(12.4668088887924,-10.,50.3352653214454));
#2560=CARTESIAN_POINT('',(4.79886262727547E-6,0.,85.7009605963974));
#2561=CARTESIAN_POINT('Origin',(0.000442544535028507,0.,90.3695776431675));
#2562=CARTESIAN_POINT('',(0.,0.,85.6497800748447));
#2563=CARTESIAN_POINT('',(0.,-10.,85.6497800748447));
#2564=CARTESIAN_POINT('Origin',(41.9587512087457,0.,88.4276904088147));
#2565=CARTESIAN_POINT('Origin',(41.9587512087457,-10.,88.4276904088147));
#4062=UNCERTAINTY_MEASURE_WITH_UNIT(LENGTH_MEASURE(0.01),#4080,
'DISTANCE_ACCURACY_VALUE',
'Maximum model space distance between geometric entities at asserted c
onnectivities');
#4069=UNCERTAINTY_MEASURE_WITH_UNIT(LENGTH_MEASURE(0.01),#4080,
'DISTANCE_ACCURACY_VALUE',
'Maximum model space distance between geometric entities at asserted c
onnectivities');
#4072=(
GEOMETRIC_REPRESENTATION_CONTEXT(3)
GLOBAL_UNCERTAINTY_ASSIGNED_CONTEXT((#4062))
GLOBAL_UNIT_ASSIGNED_CONTEXT((#4080,#4082,#4083))
REPRESENTATION_CONTEXT('','3D')
);
#4079=(
GEOMETRIC_REPRESENTATION_CONTEXT(3)
GLOBAL_UNCERTAINTY_ASSIGNED_CONTEXT((#4069))
GLOBAL_UNIT_ASSIGNED_CONTEXT((#4080,#4082,#4083))
REPRESENTATION_CONTEXT('','3D')
);
#4080=(
LENGTH_UNIT()
NAMED_UNIT(*)
SI_UNIT(.MILLI.,.METRE.)
);
#4082=(
NAMED_UNIT(*)
PLANE_ANGLE_UNIT()
SI_UNIT($,.RADIAN.)
);
#4083=(
NAMED_UNIT(*)
SI_UNIT($,.STERADIAN.)
SOLID_ANGLE_UNIT()
);
#4086=SHAPE_DEFINITION_REPRESENTATION(#4095,#4112);
#4095=PRODUCT_DEFINITION_SHAPE('',$,#4122);
#4112=SHAPE_REPRESENTATION('',(#1619),#4072);
#4119=PRODUCT_DEFINITION_CONTEXT('part definition',#4148,'design');
#4122=PRODUCT_DEFINITION('Pawl','Pawl',#4131,#4119);
#4131=PRODUCT_DEFINITION_FORMATION('',$,#4152);
#4148=APPLICATION_CONTEXT(
'Core Data for Automotive Mechanical Design Process');
#4149=PRODUCT_CONTEXT('part definition',#4148,'mechanical');
#4152=PRODUCT('Pawl','Pawl',$,(#4149));
#4161=PRESENTATION_STYLE_ASSIGNMENT((#4165));
#4165=SURFACE_STYLE_USAGE(.BOTH.,#4169);
#4169=SURFACE_SIDE_STYLE('',(#4173));
#4173=SURFACE_STYLE_FILL_AREA(#4177);
#4177=FILL_AREA_STYLE('Stainless Steel - Polished',(#4181));
#4181=FILL_AREA_STYLE_COLOUR('Stainless Steel - Polished',#4185);
#4185=COLOUR_RGB('Stainless Steel - Polished', 0.66274510, 0.83137255, 0.94901961);
ENDSEC;
END-ISO-10303-21;
